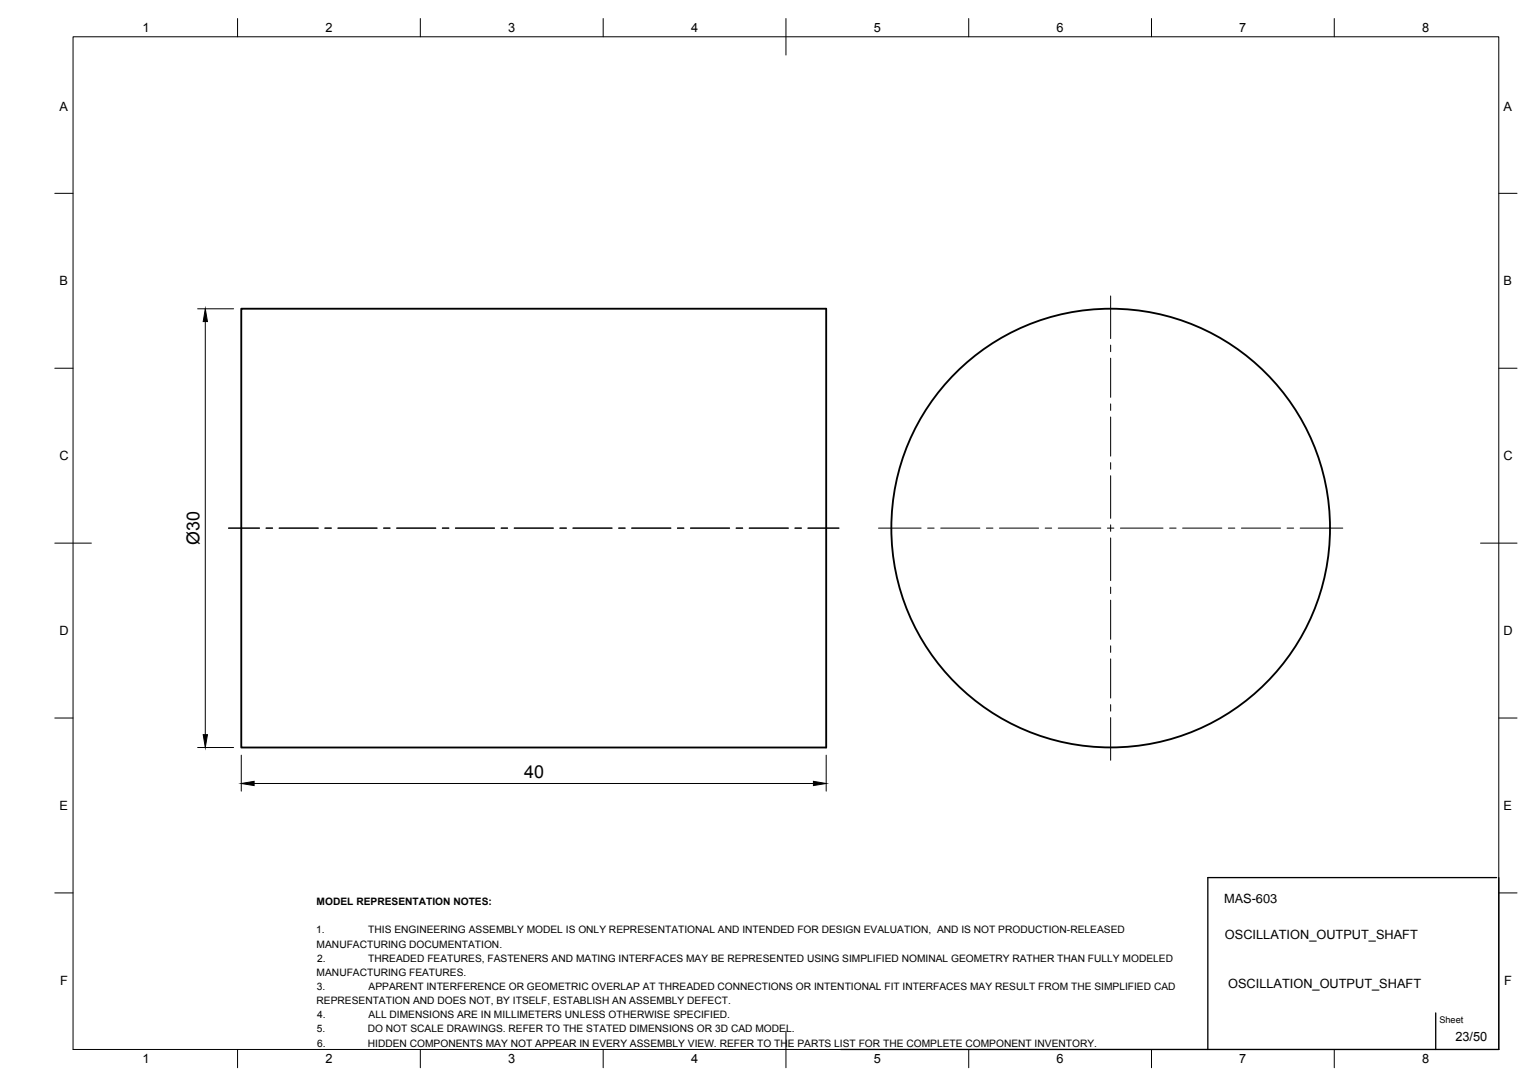
ISO-10303-21;
HEADER;
FILE_DESCRIPTION((''),'2;1');
FILE_NAME('OSCILLATION_OUTPUT_SHAFT.step','2026-10-01T22:06:14-07:00',(''),(''),'','','');
FILE_SCHEMA (('AUTOMOTIVE_DESIGN { 1 0 10303 214 3 1 1 }'));
ENDSEC;
DATA;
#10=MECHANICAL_DESIGN_GEOMETRIC_PRESENTATION_REPRESENTATION('',(#995),#50440);
#905=SHAPE_REPRESENTATION_RELATIONSHIP('SRR','None',#50637,#950) ;
#950=ADVANCED_BREP_SHAPE_REPRESENTATION('',(#1050),#50406) ;
#995=STYLED_ITEM('',(#50883),#1050) ;
#1050=MANIFOLD_SOLID_BREP('OSCILLATION_OUTPUT_SHAFT',#28662) ;
#2046=PLANE('',#30543) ;
#2047=PLANE('',#30544) ;
#3178=FACE_OUTER_BOUND('',#4919,.T.) ;
#3179=FACE_OUTER_BOUND('',#4920,.T.) ;
#3180=FACE_OUTER_BOUND('',#4921,.T.) ;
#4919=EDGE_LOOP('',(#22949,#22950,#22951,#22952)) ;
#4920=EDGE_LOOP('',(#22953)) ;
#4921=EDGE_LOOP('',(#22954)) ;
#7441=LINE('',#45889,#9913) ;
#9913=VECTOR('',#36750,1.5) ;
#11103=CIRCLE('',#30541,1.5) ;
#11104=CIRCLE('',#30542,1.5) ;
#13299=VERTEX_POINT('',#45886) ;
#13300=VERTEX_POINT('',#45888) ;
#16740=EDGE_CURVE('',#13299,#13299,#11103,.T.) ;
#16741=EDGE_CURVE('',#13299,#13300,#7441,.T.) ;
#16742=EDGE_CURVE('',#13300,#13300,#11104,.T.) ;
#22949=ORIENTED_EDGE('',*,*,#16740,.F.) ;
#22950=ORIENTED_EDGE('',*,*,#16741,.T.) ;
#22951=ORIENTED_EDGE('',*,*,#16742,.F.) ;
#22952=ORIENTED_EDGE('',*,*,#16741,.F.) ;
#22953=ORIENTED_EDGE('',*,*,#16742,.T.) ;
#22954=ORIENTED_EDGE('',*,*,#16740,.T.) ;
#26821=CYLINDRICAL_SURFACE('',#30540,1.5) ;
#27913=ADVANCED_FACE('',(#3178),#26821,.T.) ;
#27914=ADVANCED_FACE('',(#3179),#2046,.T.) ;
#27915=ADVANCED_FACE('',(#3180),#2047,.T.) ;
#28662=CLOSED_SHELL('',(#27913,#27914,#27915)) ;
#30539=AXIS2_PLACEMENT_3D('',#45884,#36744,#36745) ;
#30540=AXIS2_PLACEMENT_3D('',#45885,#36746,#36747) ;
#30541=AXIS2_PLACEMENT_3D('',#45887,#36748,#36749) ;
#30542=AXIS2_PLACEMENT_3D('',#45890,#36751,#36752) ;
#30543=AXIS2_PLACEMENT_3D('',#45891,#36753,#36754) ;
#30544=AXIS2_PLACEMENT_3D('',#45892,#36755,#36756) ;
#36744=DIRECTION('axis',(0.,0.,1.)) ;
#36745=DIRECTION('refdir',(1.,0.,0.)) ;
#36746=DIRECTION('center_axis',(0.,1.,0.)) ;
#36747=DIRECTION('ref_axis',(1.,0.,0.)) ;
#36748=DIRECTION('center_axis',(0.,1.,0.)) ;
#36749=DIRECTION('ref_axis',(1.,0.,0.)) ;
#36750=DIRECTION('',(0.,-1.,0.)) ;
#36751=DIRECTION('center_axis',(0.,-1.,0.)) ;
#36752=DIRECTION('ref_axis',(1.,0.,0.)) ;
#36753=DIRECTION('center_axis',(0.,-1.,0.)) ;
#36754=DIRECTION('ref_axis',(-1.,0.,0.)) ;
#36755=DIRECTION('center_axis',(0.,1.,0.)) ;
#36756=DIRECTION('ref_axis',(1.,0.,0.)) ;
#45884=CARTESIAN_POINT('',(0.,0.,0.)) ;
#45885=CARTESIAN_POINT('Origin',(0.,-12.,37.)) ;
#45886=CARTESIAN_POINT('',(-1.5,-10.,37.)) ;
#45887=CARTESIAN_POINT('Origin',(0.,-10.,37.)) ;
#45888=CARTESIAN_POINT('',(-1.5,-14.,37.)) ;
#45889=CARTESIAN_POINT('',(-1.5,-12.,37.)) ;
#45890=CARTESIAN_POINT('Origin',(0.,-14.,37.)) ;
#45891=CARTESIAN_POINT('Origin',(0.,-14.,37.)) ;
#45892=CARTESIAN_POINT('Origin',(0.,-10.,37.)) ;
#50353=UNCERTAINTY_MEASURE_WITH_UNIT(LENGTH_MEASURE(0.001),#50441,
'DISTANCE_ACCURACY_VALUE',
'Maximum model space distance between geometric entities at asserted c
onnectivities') ;
#50387=UNCERTAINTY_MEASURE_WITH_UNIT(LENGTH_MEASURE(0.001),#50441,
'DISTANCE_ACCURACY_VALUE',
'Maximum model space distance between geometric entities at asserted c
onnectivities') ;
#50406=(
GEOMETRIC_REPRESENTATION_CONTEXT(3)
GLOBAL_UNCERTAINTY_ASSIGNED_CONTEXT((#50353))
GLOBAL_UNIT_ASSIGNED_CONTEXT((#50441,#50443,#50444))
REPRESENTATION_CONTEXT('','3D')
) ;
#50440=(
GEOMETRIC_REPRESENTATION_CONTEXT(3)
GLOBAL_UNCERTAINTY_ASSIGNED_CONTEXT((#50387))
GLOBAL_UNIT_ASSIGNED_CONTEXT((#50441,#50443,#50444))
REPRESENTATION_CONTEXT('','3D')
) ;
#50441=(
LENGTH_UNIT()
NAMED_UNIT(*)
SI_UNIT(.CENTI.,.METRE.)
) ;
#50443=(
NAMED_UNIT(*)
PLANE_ANGLE_UNIT()
SI_UNIT($,.RADIAN.)
) ;
#50444=(
NAMED_UNIT(*)
SI_UNIT($,.STERADIAN.)
SOLID_ANGLE_UNIT()
) ;
#50463=SHAPE_DEFINITION_REPRESENTATION(#50529,#50637) ;
#50529=PRODUCT_DEFINITION_SHAPE('',$,#50690) ;
#50637=SHAPE_REPRESENTATION('',(#30539),#50406) ;
#50671=PRODUCT_DEFINITION_CONTEXT('part definition',#50829,'design') ;
#50690=PRODUCT_DEFINITION('OSCILLATION_OUTPUT_SHAFT',
'OSCILLATION_OUTPUT_SHAFT',#50742,#50671) ;
#50742=PRODUCT_DEFINITION_FORMATION('',$,#50849) ;
#50829=APPLICATION_CONTEXT(
'Core Data for Automotive Mechanical Design Process') ;
#50830=PRODUCT_CONTEXT('part definition',#50829,'mechanical') ;
#50849=PRODUCT('OSCILLATION_OUTPUT_SHAFT','OSCILLATION_OUTPUT_SHAFT',$,(#50830)) ;
#50883=PRESENTATION_STYLE_ASSIGNMENT((#50890)) ;
#50890=SURFACE_STYLE_USAGE(.BOTH.,#50897) ;
#50897=SURFACE_SIDE_STYLE('',(#50904)) ;
#50904=SURFACE_STYLE_FILL_AREA(#50911) ;
#50911=FILL_AREA_STYLE('Steel - Satin',(#50918)) ;
#50918=FILL_AREA_STYLE_COLOUR('Steel - Satin',#50925) ;
#50925=COLOUR_RGB('Steel - Satin', 0.31764706, 0.68627451, 0.89019608) ;
ENDSEC;
END-ISO-10303-21;
